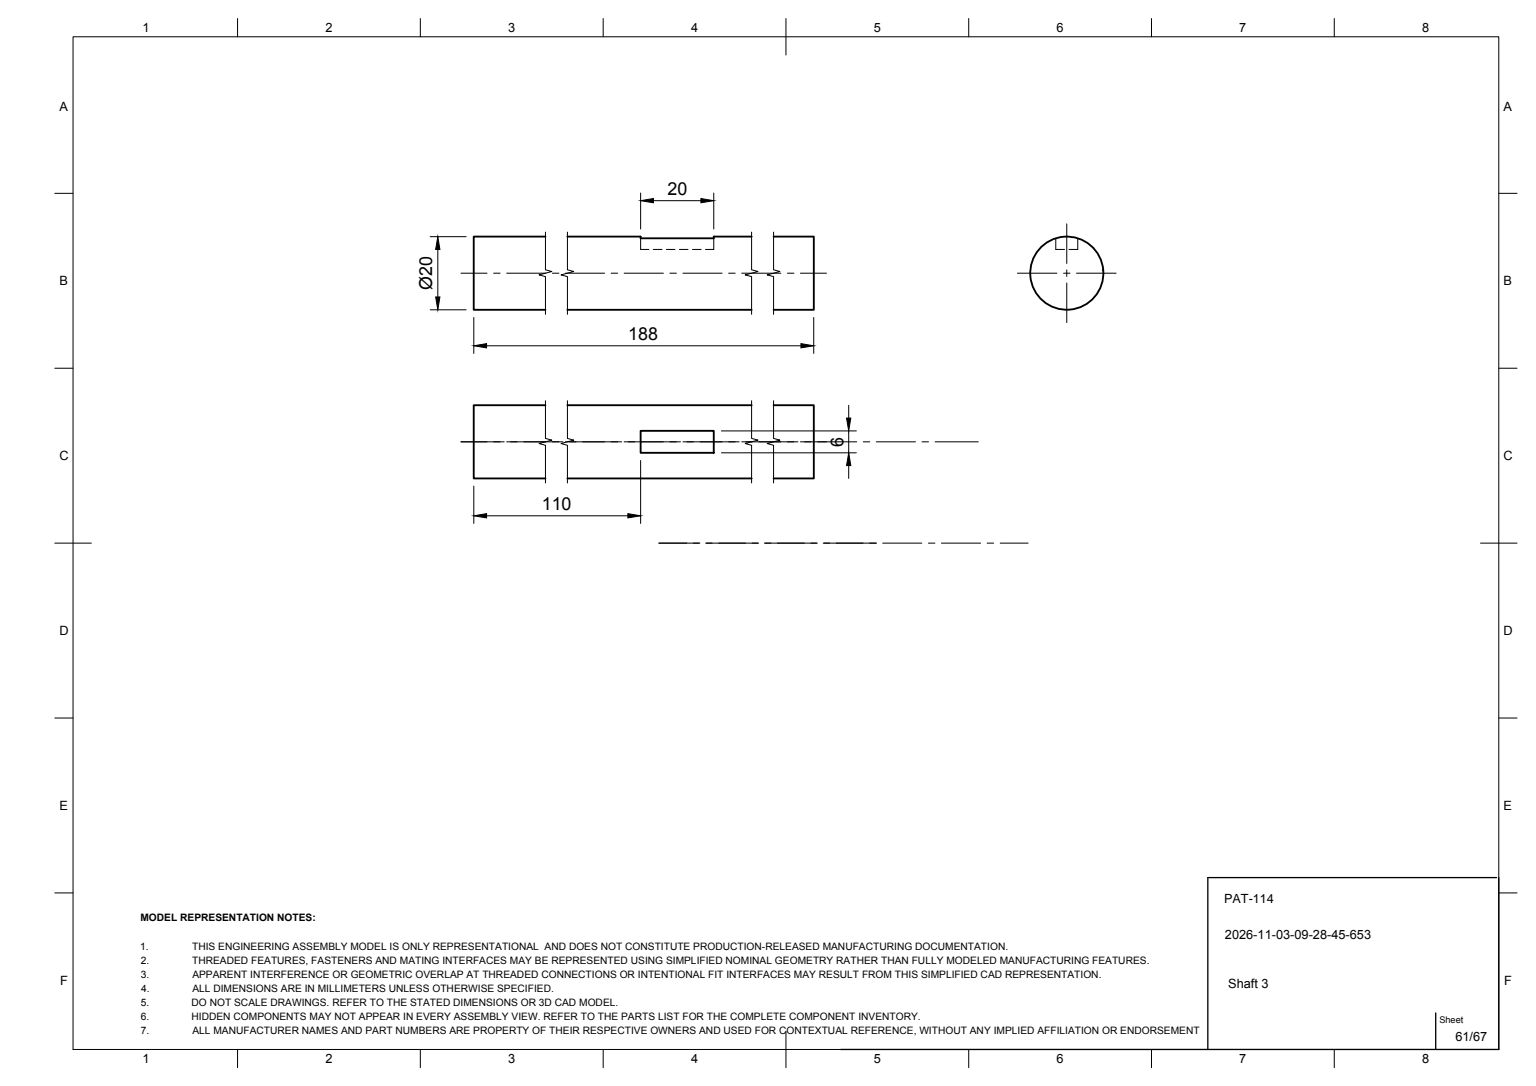
ISO-10303-21;
HEADER;
/* Generated by software containing ST-Developer
 * from STEP Tools, Inc. (www.steptools.com) 
 */

FILE_DESCRIPTION(
/* description */ ('Two-stage gear reducer in split housing'),
/* implementation_level */ '2;1');

FILE_NAME(
/* name */ 'Shaft 3.step',
/* time_stamp */ '2026-10-28T03:22:31-07:00',
/* author */ (''),
/* organization */ (''),
/* preprocessor_version */ 'ST-DEVELOPER v20.2',
/* originating_system */ 'Autodesk Translation Framework v15.17.0.0',
/* authorisation */ '');

FILE_SCHEMA (('AUTOMOTIVE_DESIGN { 1 0 10303 214 3 1 1 }'));
ENDSEC;

DATA;
#10=MECHANICAL_DESIGN_GEOMETRIC_PRESENTATION_REPRESENTATION('',(#1295),#73366);
#1168=SHAPE_REPRESENTATION_RELATIONSHIP('SRR','None',#73660,#1224);
#1224=ADVANCED_BREP_SHAPE_REPRESENTATION('',(#1364),#73356);
#1295=STYLED_ITEM('',(#73988),#1364);
#1364=MANIFOLD_SOLID_BREP('Body1',#16185);
#1581=FACE_BOUND('',#3813,.T.);
#1914=PLANE('',#18139);
#1915=PLANE('',#18140);
#1916=PLANE('',#18142);
#1917=PLANE('',#18143);
#1918=PLANE('',#18144);
#1919=PLANE('',#18149);
#1920=PLANE('',#18150);
#2687=FACE_OUTER_BOUND('',#3807,.T.);
#2688=FACE_OUTER_BOUND('',#3808,.T.);
#2689=FACE_OUTER_BOUND('',#3809,.T.);
#2690=FACE_OUTER_BOUND('',#3810,.T.);
#2691=FACE_OUTER_BOUND('',#3811,.T.);
#2692=FACE_OUTER_BOUND('',#3812,.T.);
#2693=FACE_OUTER_BOUND('',#3814,.T.);
#2694=FACE_OUTER_BOUND('',#3815,.T.);
#3807=EDGE_LOOP('',(#13677,#13678,#13679,#13680));
#3808=EDGE_LOOP('',(#13681,#13682,#13683,#13684));
#3809=EDGE_LOOP('',(#13685,#13686,#13687,#13688));
#3810=EDGE_LOOP('',(#13689,#13690,#13691,#13692));
#3811=EDGE_LOOP('',(#13693,#13694,#13695,#13696));
#3812=EDGE_LOOP('',(#13697,#13698,#13699,#13700));
#3813=EDGE_LOOP('',(#13701,#13702,#13703,#13704));
#3814=EDGE_LOOP('',(#13705));
#3815=EDGE_LOOP('',(#13706));
#4835=LINE('',#49260,#5859);
#4836=LINE('',#49262,#5860);
#4837=LINE('',#49264,#5861);
#4838=LINE('',#49265,#5862);
#4839=LINE('',#49270,#5863);
#4840=LINE('',#49271,#5864);
#4841=LINE('',#49274,#5865);
#4842=LINE('',#49276,#5866);
#4843=LINE('',#49277,#5867);
#4844=LINE('',#49279,#5868);
#4845=LINE('',#49286,#5869);
#5859=VECTOR('',#21893,1.);
#5860=VECTOR('',#21894,1.);
#5861=VECTOR('',#21895,1.);
#5862=VECTOR('',#21896,1.);
#5863=VECTOR('',#21901,1.);
#5864=VECTOR('',#21902,1.);
#5865=VECTOR('',#21905,1.);
#5866=VECTOR('',#21906,1.);
#5867=VECTOR('',#21907,1.);
#5868=VECTOR('',#21910,1.);
#5869=VECTOR('',#21919,1.);
#6702=CIRCLE('',#18141,1.);
#6703=CIRCLE('',#18145,1.);
#6704=CIRCLE('',#18147,1.);
#6705=CIRCLE('',#18148,1.);
#7897=VERTEX_POINT('',#49258);
#7898=VERTEX_POINT('',#49259);
#7899=VERTEX_POINT('',#49261);
#7900=VERTEX_POINT('',#49263);
#7901=VERTEX_POINT('',#49267);
#7902=VERTEX_POINT('',#49269);
#7903=VERTEX_POINT('',#49273);
#7904=VERTEX_POINT('',#49275);
#7905=VERTEX_POINT('',#49283);
#7906=VERTEX_POINT('',#49285);
#9892=EDGE_CURVE('',#7897,#7898,#4835,.T.);
#9893=EDGE_CURVE('',#7897,#7899,#4836,.T.);
#9894=EDGE_CURVE('',#7900,#7899,#4837,.T.);
#9895=EDGE_CURVE('',#7900,#7898,#4838,.T.);
#9896=EDGE_CURVE('',#7898,#7901,#6702,.T.);
#9897=EDGE_CURVE('',#7902,#7900,#4839,.T.);
#9898=EDGE_CURVE('',#7901,#7902,#4840,.T.);
#9899=EDGE_CURVE('',#7901,#7903,#4841,.T.);
#9900=EDGE_CURVE('',#7902,#7904,#4842,.T.);
#9901=EDGE_CURVE('',#7904,#7903,#4843,.T.);
#9902=EDGE_CURVE('',#7899,#7904,#4844,.T.);
#9903=EDGE_CURVE('',#7903,#7897,#6703,.T.);
#9904=EDGE_CURVE('',#7905,#7905,#6704,.T.);
#9905=EDGE_CURVE('',#7905,#7906,#4845,.T.);
#9906=EDGE_CURVE('',#7906,#7906,#6705,.T.);
#13677=ORIENTED_EDGE('',*,*,#9892,.F.);
#13678=ORIENTED_EDGE('',*,*,#9893,.T.);
#13679=ORIENTED_EDGE('',*,*,#9894,.F.);
#13680=ORIENTED_EDGE('',*,*,#9895,.T.);
#13681=ORIENTED_EDGE('',*,*,#9896,.F.);
#13682=ORIENTED_EDGE('',*,*,#9895,.F.);
#13683=ORIENTED_EDGE('',*,*,#9897,.F.);
#13684=ORIENTED_EDGE('',*,*,#9898,.F.);
#13685=ORIENTED_EDGE('',*,*,#9899,.F.);
#13686=ORIENTED_EDGE('',*,*,#9898,.T.);
#13687=ORIENTED_EDGE('',*,*,#9900,.T.);
#13688=ORIENTED_EDGE('',*,*,#9901,.T.);
#13689=ORIENTED_EDGE('',*,*,#9897,.T.);
#13690=ORIENTED_EDGE('',*,*,#9894,.T.);
#13691=ORIENTED_EDGE('',*,*,#9902,.T.);
#13692=ORIENTED_EDGE('',*,*,#9900,.F.);
#13693=ORIENTED_EDGE('',*,*,#9903,.F.);
#13694=ORIENTED_EDGE('',*,*,#9901,.F.);
#13695=ORIENTED_EDGE('',*,*,#9902,.F.);
#13696=ORIENTED_EDGE('',*,*,#9893,.F.);
#13697=ORIENTED_EDGE('',*,*,#9904,.F.);
#13698=ORIENTED_EDGE('',*,*,#9905,.T.);
#13699=ORIENTED_EDGE('',*,*,#9906,.T.);
#13700=ORIENTED_EDGE('',*,*,#9905,.F.);
#13701=ORIENTED_EDGE('',*,*,#9899,.T.);
#13702=ORIENTED_EDGE('',*,*,#9903,.T.);
#13703=ORIENTED_EDGE('',*,*,#9892,.T.);
#13704=ORIENTED_EDGE('',*,*,#9896,.T.);
#13705=ORIENTED_EDGE('',*,*,#9904,.T.);
#13706=ORIENTED_EDGE('',*,*,#9906,.F.);
#15151=CYLINDRICAL_SURFACE('',#18146,1.);
#15894=ADVANCED_FACE('',(#2687),#1914,.F.);
#15895=ADVANCED_FACE('',(#2688),#1915,.T.);
#15896=ADVANCED_FACE('',(#2689),#1916,.F.);
#15897=ADVANCED_FACE('',(#2690),#1917,.F.);
#15898=ADVANCED_FACE('',(#2691),#1918,.F.);
#15899=ADVANCED_FACE('',(#2692,#1581),#15151,.T.);
#15900=ADVANCED_FACE('',(#2693),#1919,.T.);
#15901=ADVANCED_FACE('',(#2694),#1920,.F.);
#16185=CLOSED_SHELL('',(#15894,#15895,#15896,#15897,#15898,#15899,#15900,
#15901));
#18138=AXIS2_PLACEMENT_3D('',#49256,#21889,#21890);
#18139=AXIS2_PLACEMENT_3D('',#49257,#21891,#21892);
#18140=AXIS2_PLACEMENT_3D('',#49266,#21897,#21898);
#18141=AXIS2_PLACEMENT_3D('',#49268,#21899,#21900);
#18142=AXIS2_PLACEMENT_3D('',#49272,#21903,#21904);
#18143=AXIS2_PLACEMENT_3D('',#49278,#21908,#21909);
#18144=AXIS2_PLACEMENT_3D('',#49280,#21911,#21912);
#18145=AXIS2_PLACEMENT_3D('',#49281,#21913,#21914);
#18146=AXIS2_PLACEMENT_3D('',#49282,#21915,#21916);
#18147=AXIS2_PLACEMENT_3D('',#49284,#21917,#21918);
#18148=AXIS2_PLACEMENT_3D('',#49287,#21920,#21921);
#18149=AXIS2_PLACEMENT_3D('',#49288,#21922,#21923);
#18150=AXIS2_PLACEMENT_3D('',#49289,#21924,#21925);
#21889=DIRECTION('axis',(0.,0.,1.));
#21890=DIRECTION('refdir',(1.,0.,0.));
#21891=DIRECTION('center_axis',(-0.996917333733128,0.,0.0784590957278455));
#21892=DIRECTION('ref_axis',(0.0784590957278455,0.,0.996917333733128));
#21893=DIRECTION('',(0.,-1.,0.));
#21894=DIRECTION('',(0.0784590957278455,0.,0.996917333733128));
#21895=DIRECTION('',(0.,1.,0.));
#21896=DIRECTION('',(-0.0784590957278455,0.,-0.996917333733128));
#21897=DIRECTION('center_axis',(0.,1.,0.));
#21898=DIRECTION('ref_axis',(1.,0.,0.));
#21899=DIRECTION('center_axis',(0.,-1.,0.));
#21900=DIRECTION('ref_axis',(1.,0.,0.));
#21901=DIRECTION('',(-0.996917333733128,0.,0.0784590957278476));
#21902=DIRECTION('',(0.0784590957278442,0.,0.996917333733128));
#21903=DIRECTION('center_axis',(0.996917333733128,0.,-0.0784590957278442));
#21904=DIRECTION('ref_axis',(-0.0784590957278442,0.,-0.996917333733128));
#21905=DIRECTION('',(0.,1.,0.));
#21906=DIRECTION('',(0.,1.,0.));
#21907=DIRECTION('',(-0.0784590957278442,0.,-0.996917333733128));
#21908=DIRECTION('center_axis',(0.0784590957278476,0.,0.996917333733128));
#21909=DIRECTION('ref_axis',(0.996917333733128,0.,-0.0784590957278476));
#21910=DIRECTION('',(0.996917333733128,0.,-0.0784590957278476));
#21911=DIRECTION('center_axis',(0.,1.,0.));
#21912=DIRECTION('ref_axis',(0.,0.,1.));
#21913=DIRECTION('center_axis',(0.,1.,0.));
#21914=DIRECTION('ref_axis',(1.,0.,0.));
#21915=DIRECTION('center_axis',(0.,1.,0.));
#21916=DIRECTION('ref_axis',(1.,0.,0.));
#21917=DIRECTION('center_axis',(0.,1.,0.));
#21918=DIRECTION('ref_axis',(1.,0.,0.));
#21919=DIRECTION('',(0.,-1.,0.));
#21920=DIRECTION('center_axis',(0.,1.,0.));
#21921=DIRECTION('ref_axis',(1.,0.,0.));
#21922=DIRECTION('center_axis',(0.,1.,0.));
#21923=DIRECTION('ref_axis',(1.,0.,0.));
#21924=DIRECTION('center_axis',(0.,1.,0.));
#21925=DIRECTION('ref_axis',(1.,0.,0.));
#49256=CARTESIAN_POINT('',(0.,0.,0.));
#49257=CARTESIAN_POINT('Origin',(11.5440066084244,1.6,8.0297030612521));
#49258=CARTESIAN_POINT('',(11.6260795927575,3.6,9.07253920349826));
#49259=CARTESIAN_POINT('',(11.6260795927575,1.6,9.07253920349826));
#49260=CARTESIAN_POINT('',(11.6260795927575,-9.4,9.07253920349826));
#49261=CARTESIAN_POINT('',(11.649926387657,3.6,9.37554146179182));
#49262=CARTESIAN_POINT('',(11.649926387657,3.6,9.37554146179182));
#49263=CARTESIAN_POINT('',(11.649926387657,1.6,9.37554146179182));
#49264=CARTESIAN_POINT('',(11.649926387657,1.6,9.37554146179182));
#49265=CARTESIAN_POINT('',(11.649926387657,1.6,9.37554146179182));
#49266=CARTESIAN_POINT('Origin',(11.8960416981606,1.6,8.67908453280361));
#49267=CARTESIAN_POINT('',(12.2242299929974,1.6,9.02546374606156));
#49268=CARTESIAN_POINT('Origin',(12.,1.6,10.));
#49269=CARTESIAN_POINT('',(12.2480767878968,1.6,9.32846600435511));
#49270=CARTESIAN_POINT('',(12.2480767878968,1.6,9.32846600435511));
#49271=CARTESIAN_POINT('',(12.1421570086642,1.6,7.98262760381539));
#49272=CARTESIAN_POINT('Origin',(12.2480767878968,1.6,9.32846600435511));
#49273=CARTESIAN_POINT('',(12.2242299929974,3.6,9.02546374606156));
#49274=CARTESIAN_POINT('',(12.2242299929974,-9.4,9.02546374606156));
#49275=CARTESIAN_POINT('',(12.2480767878968,3.6,9.32846600435511));
#49276=CARTESIAN_POINT('',(12.2480767878968,1.6,9.32846600435511));
#49277=CARTESIAN_POINT('',(12.1421570086642,3.6,7.98262760381539));
#49278=CARTESIAN_POINT('Origin',(11.649926387657,1.6,9.37554146179182));
#49279=CARTESIAN_POINT('',(12.2480767878968,3.6,9.32846600435511));
#49280=CARTESIAN_POINT('Origin',(11.8960416981606,3.6,8.67908453280361));
#49281=CARTESIAN_POINT('Origin',(12.,3.6,10.));
#49282=CARTESIAN_POINT('Origin',(12.,-9.4,10.));
#49283=CARTESIAN_POINT('',(11.,9.4,10.));
#49284=CARTESIAN_POINT('Origin',(12.,9.4,10.));
#49285=CARTESIAN_POINT('',(11.,-9.4,10.));
#49286=CARTESIAN_POINT('',(11.,-9.4,10.));
#49287=CARTESIAN_POINT('Origin',(12.,-9.4,10.));
#49288=CARTESIAN_POINT('Origin',(12.,9.4,10.));
#49289=CARTESIAN_POINT('Origin',(12.,-9.4,10.));
#73292=UNCERTAINTY_MEASURE_WITH_UNIT(LENGTH_MEASURE(0.001),#73367,
'DISTANCE_ACCURACY_VALUE',
'Maximum model space distance between geometric entities at asserted c
onnectivities');
#73302=UNCERTAINTY_MEASURE_WITH_UNIT(LENGTH_MEASURE(0.001),#73367,
'DISTANCE_ACCURACY_VALUE',
'Maximum model space distance between geometric entities at asserted c
onnectivities');
#73356=(
GEOMETRIC_REPRESENTATION_CONTEXT(3)
GLOBAL_UNCERTAINTY_ASSIGNED_CONTEXT((#73292))
GLOBAL_UNIT_ASSIGNED_CONTEXT((#73367,#73369,#73370))
REPRESENTATION_CONTEXT('','3D')
);
#73366=(
GEOMETRIC_REPRESENTATION_CONTEXT(3)
GLOBAL_UNCERTAINTY_ASSIGNED_CONTEXT((#73302))
GLOBAL_UNIT_ASSIGNED_CONTEXT((#73367,#73369,#73370))
REPRESENTATION_CONTEXT('','3D')
);
#73367=(
LENGTH_UNIT()
NAMED_UNIT(*)
SI_UNIT(.CENTI.,.METRE.)
);
#73369=(
NAMED_UNIT(*)
PLANE_ANGLE_UNIT()
SI_UNIT($,.RADIAN.)
);
#73370=(
NAMED_UNIT(*)
SI_UNIT($,.STERADIAN.)
SOLID_ANGLE_UNIT()
);
#73424=SHAPE_DEFINITION_REPRESENTATION(#73557,#73660);
#73557=PRODUCT_DEFINITION_SHAPE('',$,#73724);
#73660=SHAPE_REPRESENTATION('',(#18138),#73356);
#73670=PRODUCT_DEFINITION_CONTEXT('part definition',#73861,'design');
#73724=PRODUCT_DEFINITION('Shaft 3','Shaft 3',#73787,#73670);
#73787=PRODUCT_DEFINITION_FORMATION('',$,#73916);
#73861=APPLICATION_CONTEXT(
'Core Data for Automotive Mechanical Design Process');
#73862=PRODUCT_CONTEXT('part definition',#73861,'mechanical');
#73916=PRODUCT('Shaft 3','Shaft 3','Shaft 3',(#73862));
#73982=COLOUR_RGB('Grey',0.48,0.52,0.57);
#73983=FILL_AREA_STYLE_COLOUR('',#73982);
#73984=FILL_AREA_STYLE('',(#73983));
#73985=SURFACE_STYLE_FILL_AREA(#73984);
#73986=SURFACE_SIDE_STYLE('',(#73985));
#73987=SURFACE_STYLE_USAGE(.BOTH.,#73986);
#73988=PRESENTATION_STYLE_ASSIGNMENT((#73987));
ENDSEC;
END-ISO-10303-21;
